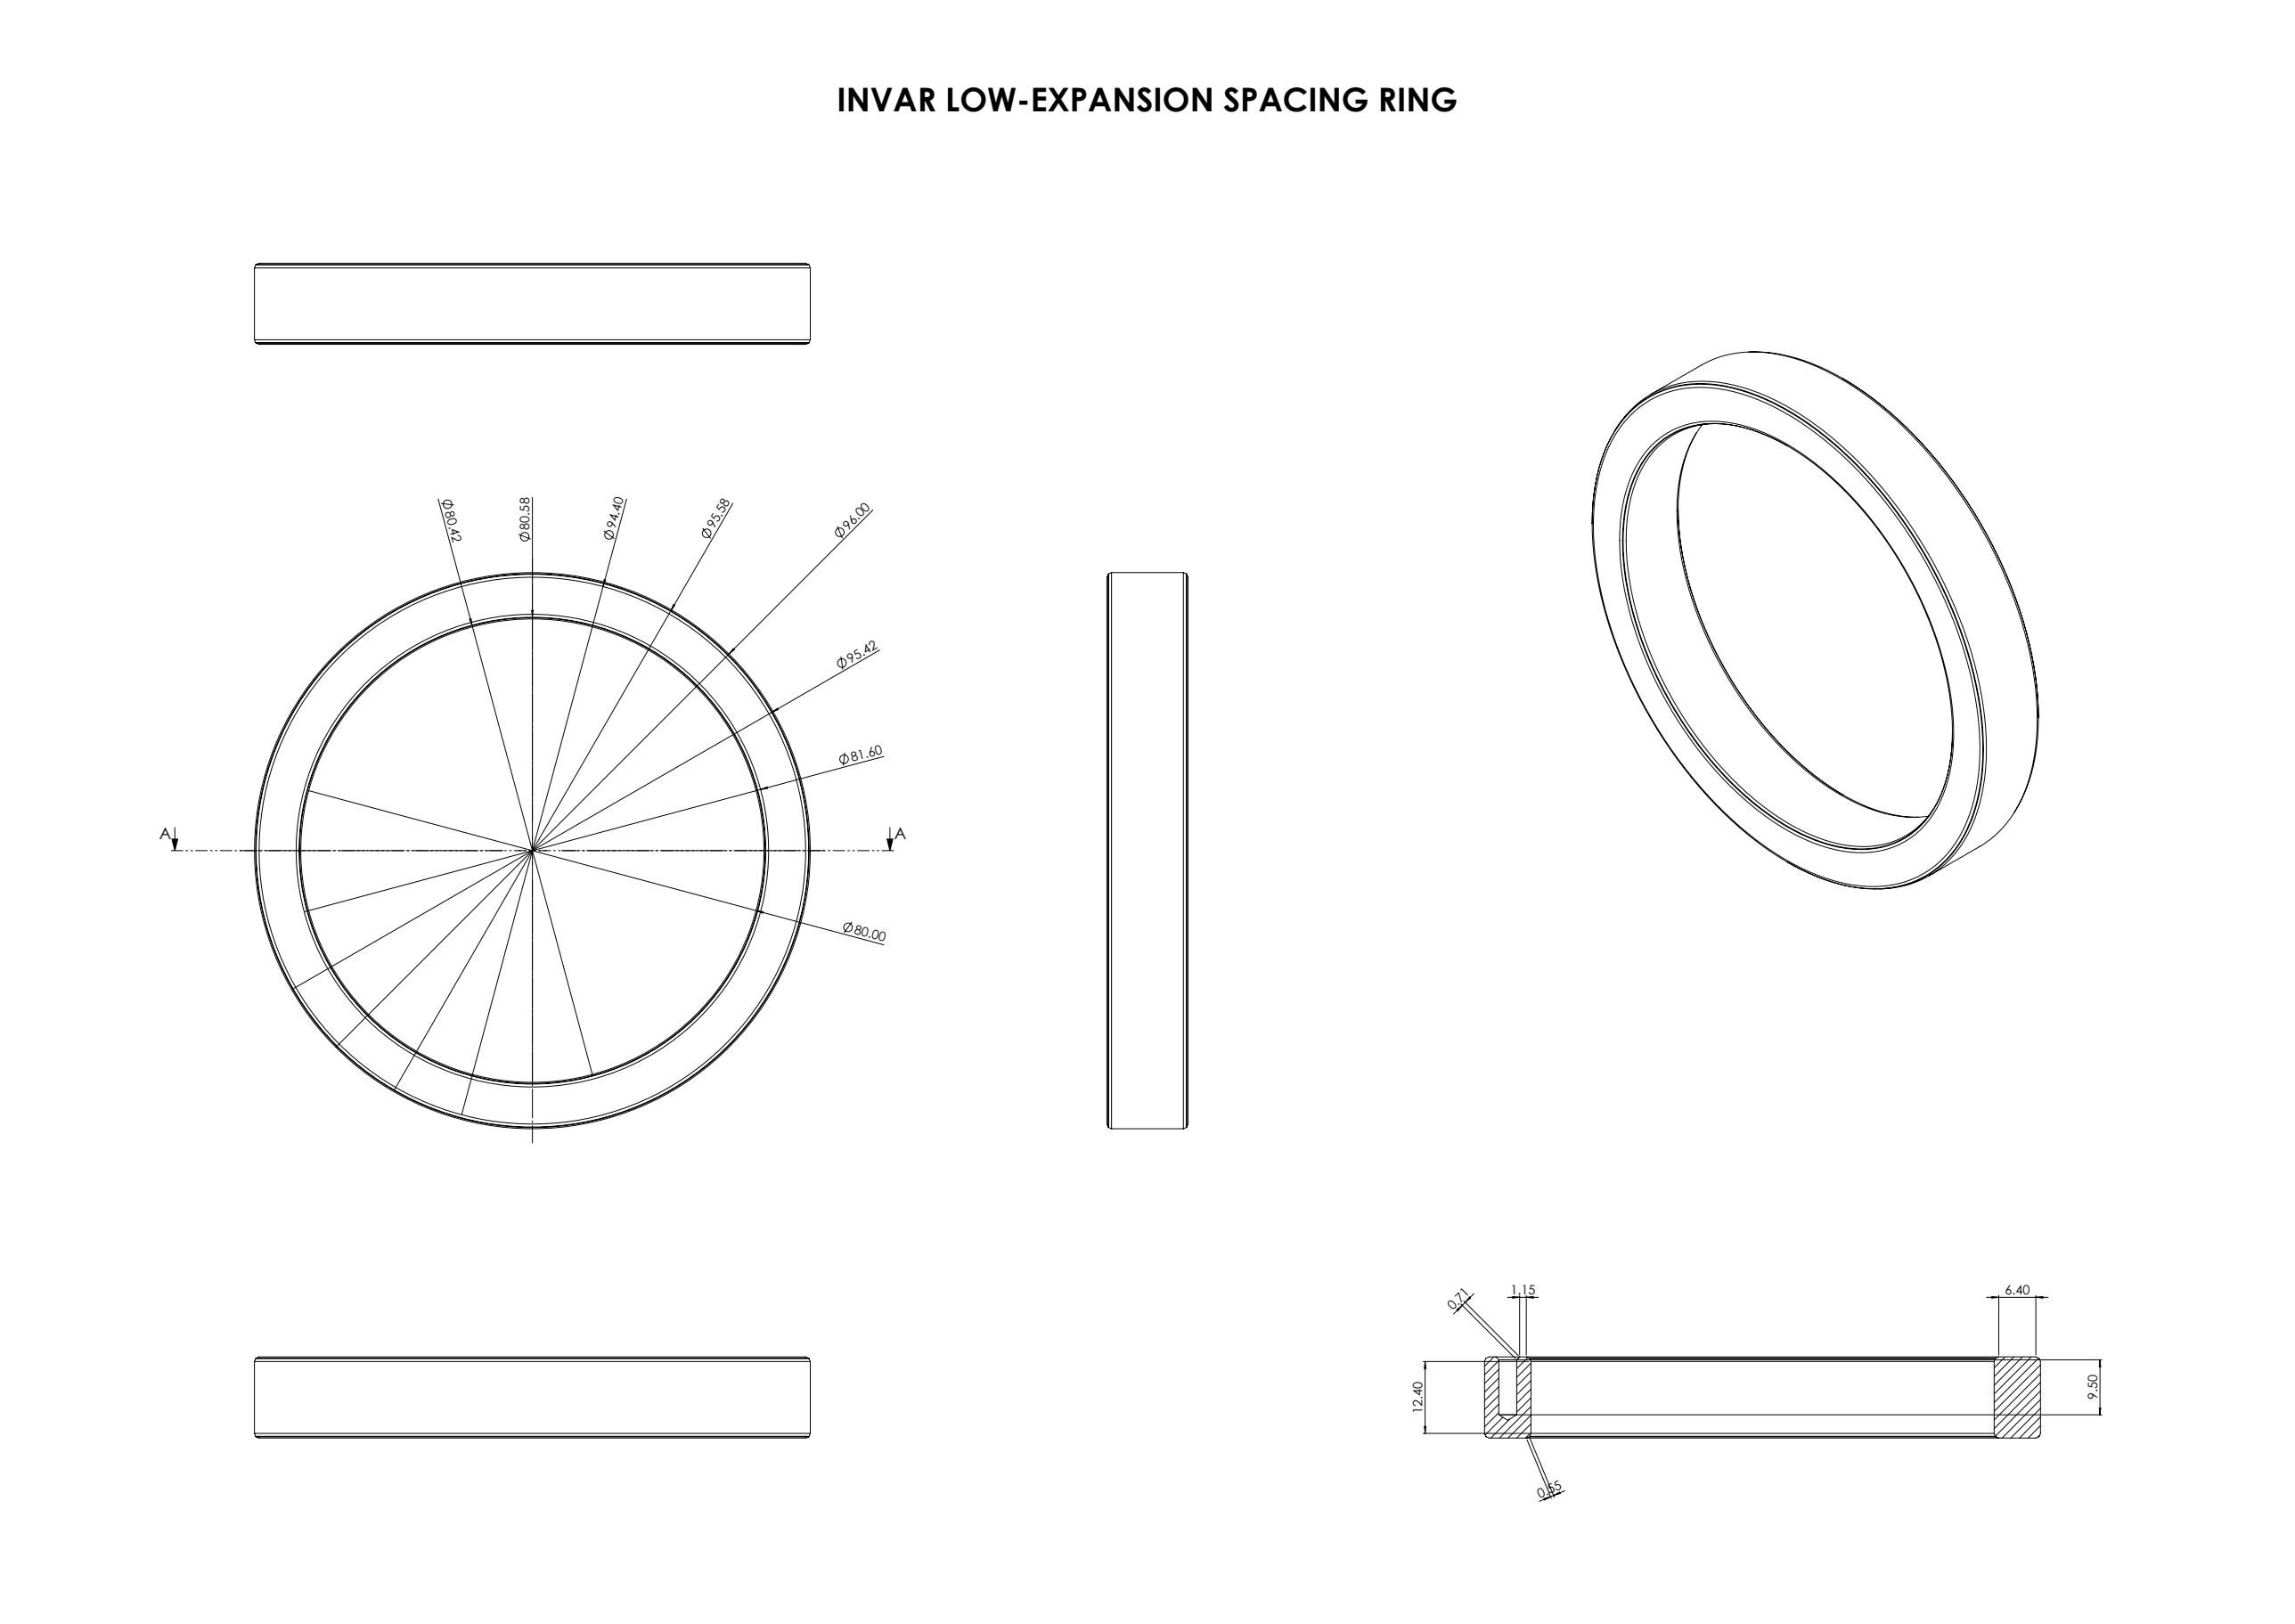
ISO-10303-21;
HEADER;
/* Generated by software containing ST-Developer
 * from STEP Tools, Inc. (www.steptools.com) 
 */

FILE_DESCRIPTION(
/* description */ (''),
/* implementation_level */ '2;1');

FILE_NAME(
/* name */ '04_Invar_Low-Expansion_Spacing_Ring.step',
/* time_stamp */ '2026-10-19T22:59:19-07:00',
/* author */ (''),
/* organization */ (''),
/* preprocessor_version */ 'ST-DEVELOPER v20.2',
/* originating_system */ 'Autodesk Translation Framework v15.15.0.0',
/* authorisation */ '');

FILE_SCHEMA (('AUTOMOTIVE_DESIGN { 1 0 10303 214 3 1 1 }'));
ENDSEC;

DATA;
#10=MECHANICAL_DESIGN_GEOMETRIC_PRESENTATION_REPRESENTATION('',(#914),#53650);
#882=SHAPE_REPRESENTATION_RELATIONSHIP('SRR','None',#53727,#898);
#898=ADVANCED_BREP_SHAPE_REPRESENTATION('',(#930),#53637);
#914=STYLED_ITEM('',(#53972),#930);
#930=MANIFOLD_SOLID_BREP('Invar Spacing Ring',#23306);
#987=CYLINDRICAL_SURFACE('',#23988,4.);
#988=CYLINDRICAL_SURFACE('',#24015,4.8);
#989=CYLINDRICAL_SURFACE('',#24025,0.155);
#990=CYLINDRICAL_SURFACE('',#24030,0.154999999999999);
#991=CYLINDRICAL_SURFACE('',#24035,0.155);
#1326=FACE_BOUND('',#3888,.T.);
#1327=FACE_BOUND('',#3889,.T.);
#1328=FACE_BOUND('',#3890,.T.);
#1329=FACE_BOUND('',#3891,.T.);
#1330=FACE_BOUND('',#3896,.T.);
#1549=PLANE('',#23999);
#1550=PLANE('',#24010);
#2504=FACE_OUTER_BOUND('',#3881,.T.);
#2505=FACE_OUTER_BOUND('',#3882,.T.);
#2506=FACE_OUTER_BOUND('',#3883,.T.);
#2507=FACE_OUTER_BOUND('',#3884,.T.);
#2508=FACE_OUTER_BOUND('',#3885,.T.);
#2509=FACE_OUTER_BOUND('',#3886,.T.);
#2510=FACE_OUTER_BOUND('',#3887,.T.);
#2511=FACE_OUTER_BOUND('',#3892,.T.);
#2512=FACE_OUTER_BOUND('',#3893,.T.);
#2513=FACE_OUTER_BOUND('',#3894,.T.);
#2514=FACE_OUTER_BOUND('',#3895,.T.);
#2515=FACE_OUTER_BOUND('',#3897,.T.);
#2516=FACE_OUTER_BOUND('',#3898,.T.);
#2517=FACE_OUTER_BOUND('',#3899,.T.);
#2518=FACE_OUTER_BOUND('',#3900,.T.);
#2519=FACE_OUTER_BOUND('',#3901,.T.);
#2520=FACE_OUTER_BOUND('',#3902,.T.);
#2521=FACE_OUTER_BOUND('',#3903,.T.);
#2522=FACE_OUTER_BOUND('',#3904,.T.);
#2523=FACE_OUTER_BOUND('',#3905,.T.);
#2524=FACE_OUTER_BOUND('',#3906,.T.);
#2525=FACE_OUTER_BOUND('',#3907,.T.);
#2526=FACE_OUTER_BOUND('',#3908,.T.);
#2527=FACE_OUTER_BOUND('',#3909,.T.);
#2528=FACE_OUTER_BOUND('',#3910,.T.);
#3881=EDGE_LOOP('',(#16211,#16212,#16213,#16214,#16215));
#3882=EDGE_LOOP('',(#16216,#16217,#16218,#16219,#16220,#16221));
#3883=EDGE_LOOP('',(#16222,#16223,#16224,#16225));
#3884=EDGE_LOOP('',(#16226,#16227,#16228,#16229,#16230));
#3885=EDGE_LOOP('',(#16231,#16232,#16233,#16234));
#3886=EDGE_LOOP('',(#16235,#16236,#16237,#16238));
#3887=EDGE_LOOP('',(#16239));
#3888=EDGE_LOOP('',(#16240));
#3889=EDGE_LOOP('',(#16241));
#3890=EDGE_LOOP('',(#16242));
#3891=EDGE_LOOP('',(#16243));
#3892=EDGE_LOOP('',(#16244,#16245,#16246,#16247));
#3893=EDGE_LOOP('',(#16248,#16249,#16250,#16251));
#3894=EDGE_LOOP('',(#16252,#16253,#16254,#16255));
#3895=EDGE_LOOP('',(#16256));
#3896=EDGE_LOOP('',(#16257));
#3897=EDGE_LOOP('',(#16258,#16259,#16260,#16261,#16262));
#3898=EDGE_LOOP('',(#16263,#16264,#16265,#16266,#16267,#16268));
#3899=EDGE_LOOP('',(#16269,#16270,#16271,#16272));
#3900=EDGE_LOOP('',(#16273,#16274,#16275,#16276));
#3901=EDGE_LOOP('',(#16277,#16278,#16279,#16280,#16281));
#3902=EDGE_LOOP('',(#16282,#16283,#16284));
#3903=EDGE_LOOP('',(#16285,#16286,#16287,#16288));
#3904=EDGE_LOOP('',(#16289,#16290,#16291,#16292));
#3905=EDGE_LOOP('',(#16293,#16294,#16295));
#3906=EDGE_LOOP('',(#16296,#16297,#16298,#16299));
#3907=EDGE_LOOP('',(#16300,#16301,#16302,#16303));
#3908=EDGE_LOOP('',(#16304,#16305,#16306));
#3909=EDGE_LOOP('',(#16307,#16308,#16309,#16310));
#3910=EDGE_LOOP('',(#16311,#16312,#16313,#16314));
#5278=CIRCLE('',#23985,4.0212132034356);
#5279=CIRCLE('',#23986,4.);
#5280=CIRCLE('',#23987,4.);
#5281=CIRCLE('',#23989,4.);
#5282=CIRCLE('',#23990,4.);
#5283=CIRCLE('',#23992,4.0287867965644);
#5284=CIRCLE('',#23994,4.0212132034356);
#5285=CIRCLE('',#23996,4.0287867965644);
#5286=CIRCLE('',#23998,4.08);
#5287=CIRCLE('',#24000,4.72);
#5288=CIRCLE('',#24001,0.205);
#5289=CIRCLE('',#24002,0.204999999999999);
#5290=CIRCLE('',#24003,0.205);
#5291=CIRCLE('',#24005,4.7712132034356);
#5292=CIRCLE('',#24007,4.7787867965644);
#5293=CIRCLE('',#24009,4.08);
#5294=CIRCLE('',#24011,4.72);
#5295=CIRCLE('',#24013,4.8);
#5296=CIRCLE('',#24014,4.8);
#5297=CIRCLE('',#24016,4.8);
#5298=CIRCLE('',#24017,4.8);
#5299=CIRCLE('',#24019,4.7712132034356);
#5300=CIRCLE('',#24021,4.7787867965644);
#5301=CIRCLE('',#24024,0.155);
#5302=CIRCLE('',#24026,0.155);
#5303=CIRCLE('',#24029,0.154999999999999);
#5304=CIRCLE('',#24031,0.154999999999999);
#5305=CIRCLE('',#24034,0.155);
#5306=CIRCLE('',#24036,0.155);
#6209=LINE('',#32993,#8054);
#6210=LINE('',#32999,#8055);
#6211=LINE('',#33005,#8056);
#6212=LINE('',#33010,#8057);
#6213=LINE('',#33014,#8058);
#6214=LINE('',#33017,#8059);
#6215=LINE('',#33031,#8060);
#6216=LINE('',#33035,#8061);
#6217=LINE('',#33038,#8062);
#6218=LINE('',#33045,#8063);
#6219=LINE('',#33054,#8064);
#6220=LINE('',#33058,#8065);
#6221=LINE('',#33061,#8066);
#6222=LINE('',#33064,#8067);
#6223=LINE('',#33068,#8068);
#6224=LINE('',#33072,#8069);
#6225=LINE('',#33075,#8070);
#6226=LINE('',#33079,#8071);
#6227=LINE('',#33083,#8072);
#6228=LINE('',#33086,#8073);
#6229=LINE('',#33090,#8074);
#6230=LINE('',#33094,#8075);
#6231=LINE('',#33097,#8076);
#8054=VECTOR('',#26991,4.0106066017178);
#8055=VECTOR('',#26998,4.);
#8056=VECTOR('',#27005,4.025);
#8057=VECTOR('',#27012,4.0106066017178);
#8058=VECTOR('',#27017,4.025);
#8059=VECTOR('',#27020,4.0543933982822);
#8060=VECTOR('',#27037,4.7456066017178);
#8061=VECTOR('',#27042,4.775);
#8062=VECTOR('',#27045,4.0543933982822);
#8063=VECTOR('',#27054,4.7893933982822);
#8064=VECTOR('',#27065,4.8);
#8065=VECTOR('',#27070,4.7456066017178);
#8066=VECTOR('',#27073,4.775);
#8067=VECTOR('',#27078,4.7893933982822);
#8068=VECTOR('',#27081,0.0774999999999997);
#8069=VECTOR('',#27086,0.155);
#8070=VECTOR('',#27091,0.205);
#8071=VECTOR('',#27094,0.0774999999999997);
#8072=VECTOR('',#27099,0.154999999999999);
#8073=VECTOR('',#27104,0.204999999999999);
#8074=VECTOR('',#27107,0.0774999999999997);
#8075=VECTOR('',#27112,0.155);
#8076=VECTOR('',#27117,0.205);
#9871=VERTEX_POINT('',#32990);
#9872=VERTEX_POINT('',#32992);
#9873=VERTEX_POINT('',#32994);
#9874=VERTEX_POINT('',#32998);
#9875=VERTEX_POINT('',#33000);
#9876=VERTEX_POINT('',#33004);
#9877=VERTEX_POINT('',#33008);
#9878=VERTEX_POINT('',#33012);
#9879=VERTEX_POINT('',#33016);
#9880=VERTEX_POINT('',#33020);
#9881=VERTEX_POINT('',#33022);
#9882=VERTEX_POINT('',#33024);
#9883=VERTEX_POINT('',#33026);
#9884=VERTEX_POINT('',#33029);
#9885=VERTEX_POINT('',#33033);
#9886=VERTEX_POINT('',#33037);
#9887=VERTEX_POINT('',#33041);
#9888=VERTEX_POINT('',#33044);
#9889=VERTEX_POINT('',#33046);
#9890=VERTEX_POINT('',#33050);
#9891=VERTEX_POINT('',#33051);
#9892=VERTEX_POINT('',#33056);
#9893=VERTEX_POINT('',#33060);
#9894=VERTEX_POINT('',#33066);
#9895=VERTEX_POINT('',#33067);
#9896=VERTEX_POINT('',#33071);
#9897=VERTEX_POINT('',#33077);
#9898=VERTEX_POINT('',#33078);
#9899=VERTEX_POINT('',#33082);
#9900=VERTEX_POINT('',#33088);
#9901=VERTEX_POINT('',#33089);
#9902=VERTEX_POINT('',#33093);
#12283=EDGE_CURVE('',#9871,#9871,#5278,.T.);
#12284=EDGE_CURVE('',#9871,#9872,#6209,.T.);
#12285=EDGE_CURVE('',#9872,#9873,#5279,.T.);
#12286=EDGE_CURVE('',#9873,#9872,#5280,.T.);
#12287=EDGE_CURVE('',#9873,#9874,#6210,.T.);
#12288=EDGE_CURVE('',#9875,#9874,#5281,.T.);
#12289=EDGE_CURVE('',#9874,#9875,#5282,.T.);
#12290=EDGE_CURVE('',#9871,#9876,#6211,.T.);
#12291=EDGE_CURVE('',#9876,#9876,#5283,.T.);
#12292=EDGE_CURVE('',#9877,#9877,#5284,.T.);
#12293=EDGE_CURVE('',#9877,#9875,#6212,.T.);
#12294=EDGE_CURVE('',#9878,#9878,#5285,.T.);
#12295=EDGE_CURVE('',#9878,#9877,#6213,.T.);
#12296=EDGE_CURVE('',#9878,#9879,#6214,.T.);
#12297=EDGE_CURVE('',#9879,#9879,#5286,.T.);
#12298=EDGE_CURVE('',#9880,#9880,#5287,.T.);
#12299=EDGE_CURVE('',#9881,#9881,#5288,.T.);
#12300=EDGE_CURVE('',#9882,#9882,#5289,.T.);
#12301=EDGE_CURVE('',#9883,#9883,#5290,.T.);
#12302=EDGE_CURVE('',#9884,#9884,#5291,.T.);
#12303=EDGE_CURVE('',#9884,#9880,#6215,.T.);
#12304=EDGE_CURVE('',#9885,#9885,#5292,.T.);
#12305=EDGE_CURVE('',#9885,#9884,#6216,.T.);
#12306=EDGE_CURVE('',#9876,#9886,#6217,.T.);
#12307=EDGE_CURVE('',#9886,#9886,#5293,.T.);
#12308=EDGE_CURVE('',#9887,#9887,#5294,.T.);
#12309=EDGE_CURVE('',#9885,#9888,#6218,.T.);
#12310=EDGE_CURVE('',#9888,#9889,#5295,.T.);
#12311=EDGE_CURVE('',#9889,#9888,#5296,.T.);
#12312=EDGE_CURVE('',#9890,#9891,#5297,.T.);
#12313=EDGE_CURVE('',#9891,#9890,#5298,.T.);
#12314=EDGE_CURVE('',#9891,#9889,#6219,.T.);
#12315=EDGE_CURVE('',#9892,#9892,#5299,.T.);
#12316=EDGE_CURVE('',#9892,#9887,#6220,.T.);
#12317=EDGE_CURVE('',#9892,#9893,#6221,.T.);
#12318=EDGE_CURVE('',#9893,#9893,#5300,.T.);
#12319=EDGE_CURVE('',#9893,#9890,#6222,.T.);
#12320=EDGE_CURVE('',#9894,#9895,#6223,.T.);
#12321=EDGE_CURVE('',#9895,#9895,#5301,.T.);
#12322=EDGE_CURVE('',#9895,#9896,#6224,.T.);
#12323=EDGE_CURVE('',#9896,#9896,#5302,.T.);
#12324=EDGE_CURVE('',#9896,#9881,#6225,.T.);
#12325=EDGE_CURVE('',#9897,#9898,#6226,.T.);
#12326=EDGE_CURVE('',#9898,#9898,#5303,.T.);
#12327=EDGE_CURVE('',#9898,#9899,#6227,.T.);
#12328=EDGE_CURVE('',#9899,#9899,#5304,.T.);
#12329=EDGE_CURVE('',#9899,#9882,#6228,.T.);
#12330=EDGE_CURVE('',#9900,#9901,#6229,.T.);
#12331=EDGE_CURVE('',#9901,#9901,#5305,.T.);
#12332=EDGE_CURVE('',#9901,#9902,#6230,.T.);
#12333=EDGE_CURVE('',#9902,#9902,#5306,.T.);
#12334=EDGE_CURVE('',#9902,#9883,#6231,.T.);
#16211=ORIENTED_EDGE('',*,*,#12283,.T.);
#16212=ORIENTED_EDGE('',*,*,#12284,.T.);
#16213=ORIENTED_EDGE('',*,*,#12285,.T.);
#16214=ORIENTED_EDGE('',*,*,#12286,.T.);
#16215=ORIENTED_EDGE('',*,*,#12284,.F.);
#16216=ORIENTED_EDGE('',*,*,#12285,.F.);
#16217=ORIENTED_EDGE('',*,*,#12286,.F.);
#16218=ORIENTED_EDGE('',*,*,#12287,.T.);
#16219=ORIENTED_EDGE('',*,*,#12288,.F.);
#16220=ORIENTED_EDGE('',*,*,#12289,.F.);
#16221=ORIENTED_EDGE('',*,*,#12287,.F.);
#16222=ORIENTED_EDGE('',*,*,#12283,.F.);
#16223=ORIENTED_EDGE('',*,*,#12290,.T.);
#16224=ORIENTED_EDGE('',*,*,#12291,.F.);
#16225=ORIENTED_EDGE('',*,*,#12290,.F.);
#16226=ORIENTED_EDGE('',*,*,#12292,.T.);
#16227=ORIENTED_EDGE('',*,*,#12293,.T.);
#16228=ORIENTED_EDGE('',*,*,#12288,.T.);
#16229=ORIENTED_EDGE('',*,*,#12289,.T.);
#16230=ORIENTED_EDGE('',*,*,#12293,.F.);
#16231=ORIENTED_EDGE('',*,*,#12294,.F.);
#16232=ORIENTED_EDGE('',*,*,#12295,.T.);
#16233=ORIENTED_EDGE('',*,*,#12292,.F.);
#16234=ORIENTED_EDGE('',*,*,#12295,.F.);
#16235=ORIENTED_EDGE('',*,*,#12294,.T.);
#16236=ORIENTED_EDGE('',*,*,#12296,.T.);
#16237=ORIENTED_EDGE('',*,*,#12297,.T.);
#16238=ORIENTED_EDGE('',*,*,#12296,.F.);
#16239=ORIENTED_EDGE('',*,*,#12298,.F.);
#16240=ORIENTED_EDGE('',*,*,#12299,.T.);
#16241=ORIENTED_EDGE('',*,*,#12300,.T.);
#16242=ORIENTED_EDGE('',*,*,#12301,.T.);
#16243=ORIENTED_EDGE('',*,*,#12297,.F.);
#16244=ORIENTED_EDGE('',*,*,#12302,.T.);
#16245=ORIENTED_EDGE('',*,*,#12303,.T.);
#16246=ORIENTED_EDGE('',*,*,#12298,.T.);
#16247=ORIENTED_EDGE('',*,*,#12303,.F.);
#16248=ORIENTED_EDGE('',*,*,#12304,.F.);
#16249=ORIENTED_EDGE('',*,*,#12305,.T.);
#16250=ORIENTED_EDGE('',*,*,#12302,.F.);
#16251=ORIENTED_EDGE('',*,*,#12305,.F.);
#16252=ORIENTED_EDGE('',*,*,#12291,.T.);
#16253=ORIENTED_EDGE('',*,*,#12306,.T.);
#16254=ORIENTED_EDGE('',*,*,#12307,.T.);
#16255=ORIENTED_EDGE('',*,*,#12306,.F.);
#16256=ORIENTED_EDGE('',*,*,#12308,.F.);
#16257=ORIENTED_EDGE('',*,*,#12307,.F.);
#16258=ORIENTED_EDGE('',*,*,#12304,.T.);
#16259=ORIENTED_EDGE('',*,*,#12309,.T.);
#16260=ORIENTED_EDGE('',*,*,#12310,.T.);
#16261=ORIENTED_EDGE('',*,*,#12311,.T.);
#16262=ORIENTED_EDGE('',*,*,#12309,.F.);
#16263=ORIENTED_EDGE('',*,*,#12312,.F.);
#16264=ORIENTED_EDGE('',*,*,#12313,.F.);
#16265=ORIENTED_EDGE('',*,*,#12314,.T.);
#16266=ORIENTED_EDGE('',*,*,#12310,.F.);
#16267=ORIENTED_EDGE('',*,*,#12311,.F.);
#16268=ORIENTED_EDGE('',*,*,#12314,.F.);
#16269=ORIENTED_EDGE('',*,*,#12315,.T.);
#16270=ORIENTED_EDGE('',*,*,#12316,.T.);
#16271=ORIENTED_EDGE('',*,*,#12308,.T.);
#16272=ORIENTED_EDGE('',*,*,#12316,.F.);
#16273=ORIENTED_EDGE('',*,*,#12315,.F.);
#16274=ORIENTED_EDGE('',*,*,#12317,.T.);
#16275=ORIENTED_EDGE('',*,*,#12318,.F.);
#16276=ORIENTED_EDGE('',*,*,#12317,.F.);
#16277=ORIENTED_EDGE('',*,*,#12318,.T.);
#16278=ORIENTED_EDGE('',*,*,#12319,.T.);
#16279=ORIENTED_EDGE('',*,*,#12312,.T.);
#16280=ORIENTED_EDGE('',*,*,#12313,.T.);
#16281=ORIENTED_EDGE('',*,*,#12319,.F.);
#16282=ORIENTED_EDGE('',*,*,#12320,.T.);
#16283=ORIENTED_EDGE('',*,*,#12321,.T.);
#16284=ORIENTED_EDGE('',*,*,#12320,.F.);
#16285=ORIENTED_EDGE('',*,*,#12321,.F.);
#16286=ORIENTED_EDGE('',*,*,#12322,.T.);
#16287=ORIENTED_EDGE('',*,*,#12323,.T.);
#16288=ORIENTED_EDGE('',*,*,#12322,.F.);
#16289=ORIENTED_EDGE('',*,*,#12323,.F.);
#16290=ORIENTED_EDGE('',*,*,#12324,.T.);
#16291=ORIENTED_EDGE('',*,*,#12299,.F.);
#16292=ORIENTED_EDGE('',*,*,#12324,.F.);
#16293=ORIENTED_EDGE('',*,*,#12325,.T.);
#16294=ORIENTED_EDGE('',*,*,#12326,.T.);
#16295=ORIENTED_EDGE('',*,*,#12325,.F.);
#16296=ORIENTED_EDGE('',*,*,#12326,.F.);
#16297=ORIENTED_EDGE('',*,*,#12327,.T.);
#16298=ORIENTED_EDGE('',*,*,#12328,.T.);
#16299=ORIENTED_EDGE('',*,*,#12327,.F.);
#16300=ORIENTED_EDGE('',*,*,#12328,.F.);
#16301=ORIENTED_EDGE('',*,*,#12329,.T.);
#16302=ORIENTED_EDGE('',*,*,#12300,.F.);
#16303=ORIENTED_EDGE('',*,*,#12329,.F.);
#16304=ORIENTED_EDGE('',*,*,#12330,.T.);
#16305=ORIENTED_EDGE('',*,*,#12331,.T.);
#16306=ORIENTED_EDGE('',*,*,#12330,.F.);
#16307=ORIENTED_EDGE('',*,*,#12331,.F.);
#16308=ORIENTED_EDGE('',*,*,#12332,.T.);
#16309=ORIENTED_EDGE('',*,*,#12333,.T.);
#16310=ORIENTED_EDGE('',*,*,#12332,.F.);
#16311=ORIENTED_EDGE('',*,*,#12333,.F.);
#16312=ORIENTED_EDGE('',*,*,#12334,.T.);
#16313=ORIENTED_EDGE('',*,*,#12301,.F.);
#16314=ORIENTED_EDGE('',*,*,#12334,.F.);
#21902=CONICAL_SURFACE('',#23984,4.0106066017178,0.392699081698746);
#21903=CONICAL_SURFACE('',#23991,4.025,0.785398163397446);
#21904=CONICAL_SURFACE('',#23993,4.0106066017178,0.392699081698729);
#21905=CONICAL_SURFACE('',#23995,4.025,0.785398163397446);
#21906=CONICAL_SURFACE('',#23997,4.0543933982822,1.17809724509616);
#21907=CONICAL_SURFACE('',#24004,4.7456066017178,1.17809724509618);
#21908=CONICAL_SURFACE('',#24006,4.775,0.785398163397446);
#21909=CONICAL_SURFACE('',#24008,4.0543933982822,1.17809724509617);
#21910=CONICAL_SURFACE('',#24012,4.7893933982822,0.392699081698714);
#21911=CONICAL_SURFACE('',#24018,4.7456066017178,1.17809724509618);
#21912=CONICAL_SURFACE('',#24020,4.775,0.785398163397446);
#21913=CONICAL_SURFACE('',#24022,4.7893933982822,0.392699081698714);
#21914=CONICAL_SURFACE('',#24023,0.0774999999999997,1.02974425867665);
#21915=CONICAL_SURFACE('',#24027,0.205,0.785398163397449);
#21916=CONICAL_SURFACE('',#24028,0.0774999999999997,1.02974425867665);
#21917=CONICAL_SURFACE('',#24032,0.204999999999999,0.785398163397447);
#21918=CONICAL_SURFACE('',#24033,0.0774999999999997,1.02974425867665);
#21919=CONICAL_SURFACE('',#24037,0.205,0.785398163397449);
#22243=ADVANCED_FACE('',(#2504),#21902,.F.);
#22244=ADVANCED_FACE('',(#2505),#987,.F.);
#22245=ADVANCED_FACE('',(#2506),#21903,.F.);
#22246=ADVANCED_FACE('',(#2507),#21904,.F.);
#22247=ADVANCED_FACE('',(#2508),#21905,.F.);
#22248=ADVANCED_FACE('',(#2509),#21906,.F.);
#22249=ADVANCED_FACE('',(#2510,#1326,#1327,#1328,#1329),#1549,.T.);
#22250=ADVANCED_FACE('',(#2511),#21907,.T.);
#22251=ADVANCED_FACE('',(#2512),#21908,.T.);
#22252=ADVANCED_FACE('',(#2513),#21909,.F.);
#22253=ADVANCED_FACE('',(#2514,#1330),#1550,.T.);
#22254=ADVANCED_FACE('',(#2515),#21910,.T.);
#22255=ADVANCED_FACE('',(#2516),#988,.T.);
#22256=ADVANCED_FACE('',(#2517),#21911,.T.);
#22257=ADVANCED_FACE('',(#2518),#21912,.T.);
#22258=ADVANCED_FACE('',(#2519),#21913,.T.);
#22259=ADVANCED_FACE('',(#2520),#21914,.F.);
#22260=ADVANCED_FACE('',(#2521),#989,.F.);
#22261=ADVANCED_FACE('',(#2522),#21915,.F.);
#22262=ADVANCED_FACE('',(#2523),#21916,.F.);
#22263=ADVANCED_FACE('',(#2524),#990,.F.);
#22264=ADVANCED_FACE('',(#2525),#21917,.F.);
#22265=ADVANCED_FACE('',(#2526),#21918,.F.);
#22266=ADVANCED_FACE('',(#2527),#991,.F.);
#22267=ADVANCED_FACE('',(#2528),#21919,.F.);
#23306=CLOSED_SHELL('',(#22243,#22244,#22245,#22246,#22247,#22248,#22249,
#22250,#22251,#22252,#22253,#22254,#22255,#22256,#22257,#22258,#22259,#22260,
#22261,#22262,#22263,#22264,#22265,#22266,#22267));
#23983=AXIS2_PLACEMENT_3D('',#32988,#26985,#26986);
#23984=AXIS2_PLACEMENT_3D('',#32989,#26987,#26988);
#23985=AXIS2_PLACEMENT_3D('',#32991,#26989,#26990);
#23986=AXIS2_PLACEMENT_3D('',#32995,#26992,#26993);
#23987=AXIS2_PLACEMENT_3D('',#32996,#26994,#26995);
#23988=AXIS2_PLACEMENT_3D('',#32997,#26996,#26997);
#23989=AXIS2_PLACEMENT_3D('',#33001,#26999,#27000);
#23990=AXIS2_PLACEMENT_3D('',#33002,#27001,#27002);
#23991=AXIS2_PLACEMENT_3D('',#33003,#27003,#27004);
#23992=AXIS2_PLACEMENT_3D('',#33006,#27006,#27007);
#23993=AXIS2_PLACEMENT_3D('',#33007,#27008,#27009);
#23994=AXIS2_PLACEMENT_3D('',#33009,#27010,#27011);
#23995=AXIS2_PLACEMENT_3D('',#33011,#27013,#27014);
#23996=AXIS2_PLACEMENT_3D('',#33013,#27015,#27016);
#23997=AXIS2_PLACEMENT_3D('',#33015,#27018,#27019);
#23998=AXIS2_PLACEMENT_3D('',#33018,#27021,#27022);
#23999=AXIS2_PLACEMENT_3D('',#33019,#27023,#27024);
#24000=AXIS2_PLACEMENT_3D('',#33021,#27025,#27026);
#24001=AXIS2_PLACEMENT_3D('',#33023,#27027,#27028);
#24002=AXIS2_PLACEMENT_3D('',#33025,#27029,#27030);
#24003=AXIS2_PLACEMENT_3D('',#33027,#27031,#27032);
#24004=AXIS2_PLACEMENT_3D('',#33028,#27033,#27034);
#24005=AXIS2_PLACEMENT_3D('',#33030,#27035,#27036);
#24006=AXIS2_PLACEMENT_3D('',#33032,#27038,#27039);
#24007=AXIS2_PLACEMENT_3D('',#33034,#27040,#27041);
#24008=AXIS2_PLACEMENT_3D('',#33036,#27043,#27044);
#24009=AXIS2_PLACEMENT_3D('',#33039,#27046,#27047);
#24010=AXIS2_PLACEMENT_3D('',#33040,#27048,#27049);
#24011=AXIS2_PLACEMENT_3D('',#33042,#27050,#27051);
#24012=AXIS2_PLACEMENT_3D('',#33043,#27052,#27053);
#24013=AXIS2_PLACEMENT_3D('',#33047,#27055,#27056);
#24014=AXIS2_PLACEMENT_3D('',#33048,#27057,#27058);
#24015=AXIS2_PLACEMENT_3D('',#33049,#27059,#27060);
#24016=AXIS2_PLACEMENT_3D('',#33052,#27061,#27062);
#24017=AXIS2_PLACEMENT_3D('',#33053,#27063,#27064);
#24018=AXIS2_PLACEMENT_3D('',#33055,#27066,#27067);
#24019=AXIS2_PLACEMENT_3D('',#33057,#27068,#27069);
#24020=AXIS2_PLACEMENT_3D('',#33059,#27071,#27072);
#24021=AXIS2_PLACEMENT_3D('',#33062,#27074,#27075);
#24022=AXIS2_PLACEMENT_3D('',#33063,#27076,#27077);
#24023=AXIS2_PLACEMENT_3D('',#33065,#27079,#27080);
#24024=AXIS2_PLACEMENT_3D('',#33069,#27082,#27083);
#24025=AXIS2_PLACEMENT_3D('',#33070,#27084,#27085);
#24026=AXIS2_PLACEMENT_3D('',#33073,#27087,#27088);
#24027=AXIS2_PLACEMENT_3D('',#33074,#27089,#27090);
#24028=AXIS2_PLACEMENT_3D('',#33076,#27092,#27093);
#24029=AXIS2_PLACEMENT_3D('',#33080,#27095,#27096);
#24030=AXIS2_PLACEMENT_3D('',#33081,#27097,#27098);
#24031=AXIS2_PLACEMENT_3D('',#33084,#27100,#27101);
#24032=AXIS2_PLACEMENT_3D('',#33085,#27102,#27103);
#24033=AXIS2_PLACEMENT_3D('',#33087,#27105,#27106);
#24034=AXIS2_PLACEMENT_3D('',#33091,#27108,#27109);
#24035=AXIS2_PLACEMENT_3D('',#33092,#27110,#27111);
#24036=AXIS2_PLACEMENT_3D('',#33095,#27113,#27114);
#24037=AXIS2_PLACEMENT_3D('',#33096,#27115,#27116);
#26985=DIRECTION('axis',(0.,0.,1.));
#26986=DIRECTION('refdir',(1.,0.,0.));
#26987=DIRECTION('center_axis',(0.,-4.80790650449101E-15,1.));
#26988=DIRECTION('ref_axis',(-1.,3.06971386583218E-17,0.));
#26989=DIRECTION('center_axis',(0.,0.,1.));
#26990=DIRECTION('ref_axis',(-1.,6.12323399573677E-17,0.));
#26991=DIRECTION('',(-0.38268343236511,4.40680849605938E-15,-0.923879532511278));
#26992=DIRECTION('center_axis',(0.,0.,-1.));
#26993=DIRECTION('ref_axis',(-1.,0.,0.));
#26994=DIRECTION('center_axis',(0.,0.,-1.));
#26995=DIRECTION('ref_axis',(-1.,0.,0.));
#26996=DIRECTION('center_axis',(0.,0.,1.));
#26997=DIRECTION('ref_axis',(1.,0.,0.));
#26998=DIRECTION('',(0.,0.,-1.));
#26999=DIRECTION('center_axis',(0.,0.,1.));
#27000=DIRECTION('ref_axis',(-1.,0.,0.));
#27001=DIRECTION('center_axis',(0.,0.,1.));
#27002=DIRECTION('ref_axis',(-1.,0.,0.));
#27003=DIRECTION('center_axis',(0.,0.,1.));
#27004=DIRECTION('ref_axis',(-1.,0.,0.));
#27005=DIRECTION('',(0.707106781186546,-8.65956056235492E-17,0.707106781186549));
#27006=DIRECTION('center_axis',(0.,0.,-1.));
#27007=DIRECTION('ref_axis',(-1.,6.12323399573677E-17,0.));
#27008=DIRECTION('center_axis',(0.,-4.80790650449097E-15,-1.));
#27009=DIRECTION('ref_axis',(-1.,3.06971386583218E-17,0.));
#27010=DIRECTION('center_axis',(0.,0.,-1.));
#27011=DIRECTION('ref_axis',(-1.,6.12323399573677E-17,0.));
#27012=DIRECTION('',(-0.382683432365094,4.5005389041659E-15,0.923879532511285));
#27013=DIRECTION('center_axis',(0.,0.,-1.));
#27014=DIRECTION('ref_axis',(-1.,0.,0.));
#27015=DIRECTION('center_axis',(0.,0.,1.));
#27016=DIRECTION('ref_axis',(-1.,6.12323399573677E-17,0.));
#27017=DIRECTION('',(-0.707106781186546,8.65956056235492E-17,0.707106781186549));
#27018=DIRECTION('center_axis',(0.,1.16291744192215E-14,-1.));
#27019=DIRECTION('ref_axis',(-1.,3.04228054001255E-17,0.));
#27020=DIRECTION('',(0.923879532511283,4.53532798631812E-15,-0.382683432365099));
#27021=DIRECTION('center_axis',(0.,0.,-1.));
#27022=DIRECTION('ref_axis',(-1.,0.,0.));
#27023=DIRECTION('center_axis',(0.,0.,-1.));
#27024=DIRECTION('ref_axis',(-1.,0.,0.));
#27025=DIRECTION('center_axis',(0.,0.,1.));
#27026=DIRECTION('ref_axis',(-1.,0.,0.));
#27027=DIRECTION('center_axis',(0.,0.,1.));
#27028=DIRECTION('ref_axis',(-1.,0.,0.));
#27029=DIRECTION('center_axis',(0.,0.,1.));
#27030=DIRECTION('ref_axis',(-1.,0.,0.));
#27031=DIRECTION('center_axis',(0.,0.,1.));
#27032=DIRECTION('ref_axis',(-1.,0.,0.));
#27033=DIRECTION('center_axis',(0.,1.37722032303527E-14,1.));
#27034=DIRECTION('ref_axis',(-1.,-3.078137037066E-17,0.));
#27035=DIRECTION('center_axis',(0.,0.,-1.));
#27036=DIRECTION('ref_axis',(-1.,-6.12323399573677E-17,0.));
#27037=DIRECTION('',(-0.923879532511289,-5.41197489271776E-15,-0.382683432365086));
#27038=DIRECTION('center_axis',(0.,0.,1.));
#27039=DIRECTION('ref_axis',(-1.,0.,0.));
#27040=DIRECTION('center_axis',(0.,0.,1.));
#27041=DIRECTION('ref_axis',(-1.,-6.12323399573676E-17,0.));
#27042=DIRECTION('',(-0.707106781186546,-8.65956056235491E-17,-0.707106781186549));
#27043=DIRECTION('center_axis',(0.,1.16291744192216E-14,1.));
#27044=DIRECTION('ref_axis',(-1.,3.04228054001255E-17,0.));
#27045=DIRECTION('',(0.923879532511284,4.30904276386059E-15,0.382683432365097));
#27046=DIRECTION('center_axis',(0.,0.,1.));
#27047=DIRECTION('ref_axis',(-1.,0.,0.));
#27048=DIRECTION('center_axis',(0.,0.,1.));
#27049=DIRECTION('ref_axis',(1.,0.,0.));
#27050=DIRECTION('center_axis',(0.,0.,-1.));
#27051=DIRECTION('ref_axis',(-1.,0.,0.));
#27052=DIRECTION('center_axis',(0.,-5.71368862092357E-15,1.));
#27053=DIRECTION('ref_axis',(-1.,-3.05483673377054E-17,0.));
#27054=DIRECTION('',(0.382683432365081,-5.31393482200127E-15,0.923879532511291));
#27055=DIRECTION('center_axis',(0.,0.,-1.));
#27056=DIRECTION('ref_axis',(-1.,0.,0.));
#27057=DIRECTION('center_axis',(0.,0.,-1.));
#27058=DIRECTION('ref_axis',(-1.,0.,0.));
#27059=DIRECTION('center_axis',(0.,0.,1.));
#27060=DIRECTION('ref_axis',(1.,0.,0.));
#27061=DIRECTION('center_axis',(0.,0.,1.));
#27062=DIRECTION('ref_axis',(-1.,0.,0.));
#27063=DIRECTION('center_axis',(0.,0.,1.));
#27064=DIRECTION('ref_axis',(-1.,0.,0.));
#27065=DIRECTION('',(0.,0.,-1.));
#27066=DIRECTION('center_axis',(0.,1.37722032303528E-14,-1.));
#27067=DIRECTION('ref_axis',(-1.,-3.078137037066E-17,0.));
#27068=DIRECTION('center_axis',(0.,0.,1.));
#27069=DIRECTION('ref_axis',(-1.,-6.12323399573677E-17,0.));
#27070=DIRECTION('',(-0.923879532511289,-5.18568967026023E-15,0.382683432365084));
#27071=DIRECTION('center_axis',(0.,0.,-1.));
#27072=DIRECTION('ref_axis',(-1.,0.,0.));
#27073=DIRECTION('',(0.707106781186546,8.65956056235491E-17,-0.707106781186549));
#27074=DIRECTION('center_axis',(0.,0.,-1.));
#27075=DIRECTION('ref_axis',(-1.,-6.12323399573677E-17,0.));
#27076=DIRECTION('center_axis',(0.,-5.71368862092356E-15,-1.));
#27077=DIRECTION('ref_axis',(-1.,-3.05483673377054E-17,0.));
#27078=DIRECTION('',(0.38268343236508,-5.22020441389474E-15,-0.923879532511291));
#27079=DIRECTION('center_axis',(0.,0.,-1.));
#27080=DIRECTION('ref_axis',(-1.,0.,0.));
#27081=DIRECTION('',(0.857167300702112,-1.04972719113862E-16,-0.515038074910055));
#27082=DIRECTION('center_axis',(0.,0.,-1.));
#27083=DIRECTION('ref_axis',(1.,0.,0.));
#27084=DIRECTION('center_axis',(0.,0.,-1.));
#27085=DIRECTION('ref_axis',(-1.,0.,0.));
#27086=DIRECTION('',(0.,0.,-1.));
#27087=DIRECTION('center_axis',(0.,0.,-1.));
#27088=DIRECTION('ref_axis',(1.,0.,0.));
#27089=DIRECTION('center_axis',(0.,0.,-1.));
#27090=DIRECTION('ref_axis',(-1.,0.,0.));
#27091=DIRECTION('',(0.707106781186548,-8.65956056235494E-17,-0.707106781186547));
#27092=DIRECTION('center_axis',(0.,0.,-1.));
#27093=DIRECTION('ref_axis',(-1.,0.,0.));
#27094=DIRECTION('',(0.857167300702111,-1.04972719113862E-16,-0.515038074910056));
#27095=DIRECTION('center_axis',(0.,0.,-1.));
#27096=DIRECTION('ref_axis',(1.,0.,0.));
#27097=DIRECTION('center_axis',(0.,0.,-1.));
#27098=DIRECTION('ref_axis',(-1.,0.,0.));
#27099=DIRECTION('',(0.,0.,-1.));
#27100=DIRECTION('center_axis',(0.,0.,-1.));
#27101=DIRECTION('ref_axis',(1.,0.,0.));
#27102=DIRECTION('center_axis',(0.,0.,-1.));
#27103=DIRECTION('ref_axis',(-1.,0.,0.));
#27104=DIRECTION('',(0.707106781186546,-8.65956056235492E-17,-0.707106781186549));
#27105=DIRECTION('center_axis',(0.,0.,-1.));
#27106=DIRECTION('ref_axis',(-1.,0.,0.));
#27107=DIRECTION('',(0.857167300702112,-1.04972719113862E-16,-0.515038074910055));
#27108=DIRECTION('center_axis',(0.,0.,-1.));
#27109=DIRECTION('ref_axis',(1.,0.,0.));
#27110=DIRECTION('center_axis',(0.,0.,-1.));
#27111=DIRECTION('ref_axis',(-1.,0.,0.));
#27112=DIRECTION('',(0.,0.,-1.));
#27113=DIRECTION('center_axis',(0.,0.,-1.));
#27114=DIRECTION('ref_axis',(1.,0.,0.));
#27115=DIRECTION('center_axis',(0.,0.,-1.));
#27116=DIRECTION('ref_axis',(-1.,0.,0.));
#27117=DIRECTION('',(0.707106781186548,-8.65956056235494E-17,-0.707106781186547));
#32988=CARTESIAN_POINT('',(0.,0.,0.));
#32989=CARTESIAN_POINT('Origin',(0.,-1.23114146956912E-16,1.3456066017178));
#32990=CARTESIAN_POINT('',(4.0212132034356,0.,1.3712132034356));
#32991=CARTESIAN_POINT('Origin',(0.,-2.46228293913824E-16,1.3712132034356));
#32992=CARTESIAN_POINT('',(4.,-4.89858719658941E-16,1.32));
#32993=CARTESIAN_POINT('',(4.0106066017178,2.44929359829471E-16,1.3456066017178));
#32994=CARTESIAN_POINT('',(-4.,-4.89858719658941E-16,1.32));
#32995=CARTESIAN_POINT('Origin',(0.,0.,1.32));
#32996=CARTESIAN_POINT('Origin',(0.,0.,1.32));
#32997=CARTESIAN_POINT('Origin',(0.,0.,0.7));
#32998=CARTESIAN_POINT('',(-4.,-4.89858719658941E-16,0.08));
#32999=CARTESIAN_POINT('',(-4.,-4.89858719658941E-16,0.7));
#33000=CARTESIAN_POINT('',(4.,4.89858719658941E-16,0.08));
#33001=CARTESIAN_POINT('Origin',(0.,0.,0.08));
#33002=CARTESIAN_POINT('Origin',(0.,0.,0.08));
#33003=CARTESIAN_POINT('Origin',(0.,0.,1.375));
#33004=CARTESIAN_POINT('',(4.0287867965644,-9.86768170971943E-16,1.3787867965644));
#33005=CARTESIAN_POINT('',(4.025,-4.9292033665681E-16,1.375));
#33006=CARTESIAN_POINT('Origin',(0.,-2.46692042742986E-16,1.3787867965644));
#33007=CARTESIAN_POINT('Origin',(0.,-1.23114146956912E-16,0.0543933982822017));
#33008=CARTESIAN_POINT('',(4.0212132034356,-9.84913175655296E-16,0.0287867965644034));
#33009=CARTESIAN_POINT('Origin',(0.,-2.46228293913824E-16,0.0287867965644034));
#33010=CARTESIAN_POINT('',(4.0106066017178,-7.37385947657118E-16,0.0543933982822017));
#33011=CARTESIAN_POINT('Origin',(0.,0.,0.025));
#33012=CARTESIAN_POINT('',(4.0287867965644,0.,0.0212132034355969));
#33013=CARTESIAN_POINT('Origin',(0.,-2.46692042742986E-16,0.0212132034355969));
#33014=CARTESIAN_POINT('',(4.025,-4.9292033665681E-16,0.025));
#33015=CARTESIAN_POINT('Origin',(0.,-1.23346021371493E-16,0.0106066017177984));
#33016=CARTESIAN_POINT('',(4.08,-4.9965589405212E-16,0.));
#33017=CARTESIAN_POINT('',(4.0543933982822,2.4982794702606E-16,0.0106066017177984));
#33018=CARTESIAN_POINT('Origin',(0.,0.,0.));
#33019=CARTESIAN_POINT('Origin',(4.8,0.,0.));
#33020=CARTESIAN_POINT('',(4.72,5.78033289197551E-16,0.));
#33021=CARTESIAN_POINT('Origin',(0.,0.,0.));
#33022=CARTESIAN_POINT('',(2.405,-3.81051177665153,0.));
#33023=CARTESIAN_POINT('Origin',(2.2,-3.81051177665153,0.));
#33024=CARTESIAN_POINT('',(-4.195,5.63949851007356E-16,0.));
#33025=CARTESIAN_POINT('Origin',(-4.4,5.38844591624835E-16,0.));
#33026=CARTESIAN_POINT('',(2.405,3.81051177665153,0.));
#33027=CARTESIAN_POINT('Origin',(2.2,3.81051177665153,0.));
#33028=CARTESIAN_POINT('Origin',(0.,1.46076274440925E-16,0.0106066017177982));
#33029=CARTESIAN_POINT('',(4.7712132034356,0.,0.0212132034355964));
#33030=CARTESIAN_POINT('Origin',(0.,2.9215254888185E-16,0.0212132034355964));
#33031=CARTESIAN_POINT('',(4.7456066017178,8.73321742362474E-16,0.0106066017177982));
#33032=CARTESIAN_POINT('Origin',(0.,0.,0.025));
#33033=CARTESIAN_POINT('',(4.7787867965644,1.17046519084405E-15,0.0287867965644034));
#33034=CARTESIAN_POINT('Origin',(0.,2.92616297711012E-16,0.0287867965644034));
#33035=CARTESIAN_POINT('',(4.775,5.84768846592861E-16,0.025));
#33036=CARTESIAN_POINT('Origin',(0.,-1.23346021371493E-16,1.3893933982822));
#33037=CARTESIAN_POINT('',(4.08,4.9965589405212E-16,1.4));
#33038=CARTESIAN_POINT('',(4.0543933982822,-7.43212032512032E-16,1.3893933982822));
#33039=CARTESIAN_POINT('Origin',(0.,0.,1.4));
#33040=CARTESIAN_POINT('Origin',(4.,0.,1.4));
#33041=CARTESIAN_POINT('',(4.72,-5.78033289197551E-16,1.4));
#33042=CARTESIAN_POINT('Origin',(0.,0.,1.4));
#33043=CARTESIAN_POINT('Origin',(0.,1.46308148855506E-16,0.0543933982822016));
#33044=CARTESIAN_POINT('',(4.8,-5.8783046359073E-16,0.0799999999999998));
#33045=CARTESIAN_POINT('',(4.7893933982822,-2.93915231795365E-16,0.0543933982822016));
#33046=CARTESIAN_POINT('',(-4.8,-5.8783046359073E-16,0.0799999999999997));
#33047=CARTESIAN_POINT('Origin',(0.,0.,0.0799999999999998));
#33048=CARTESIAN_POINT('Origin',(0.,0.,0.0799999999999998));
#33049=CARTESIAN_POINT('Origin',(0.,0.,0.7));
#33050=CARTESIAN_POINT('',(4.8,5.8783046359073E-16,1.32));
#33051=CARTESIAN_POINT('',(-4.8,-5.8783046359073E-16,1.32));
#33052=CARTESIAN_POINT('Origin',(0.,0.,1.32));
#33053=CARTESIAN_POINT('Origin',(0.,0.,1.32));
#33054=CARTESIAN_POINT('',(-4.8,-5.8783046359073E-16,0.7));
#33055=CARTESIAN_POINT('Origin',(0.,1.46076274440925E-16,1.3893933982822));
#33056=CARTESIAN_POINT('',(4.7712132034356,1.1686101955274E-15,1.3787867965644));
#33057=CARTESIAN_POINT('Origin',(0.,2.9215254888185E-16,1.3787867965644));
#33058=CARTESIAN_POINT('',(4.7456066017178,-2.89016644598775E-16,1.3893933982822));
#33059=CARTESIAN_POINT('Origin',(0.,0.,1.375));
#33060=CARTESIAN_POINT('',(4.7787867965644,0.,1.3712132034356));
#33061=CARTESIAN_POINT('',(4.775,5.84768846592861E-16,1.375));
#33062=CARTESIAN_POINT('Origin',(0.,2.92616297711012E-16,1.3712132034356));
#33063=CARTESIAN_POINT('Origin',(0.,1.46308148855506E-16,1.3456066017178));
#33064=CARTESIAN_POINT('',(4.7893933982822,8.79147827217388E-16,1.3456066017178));
#33065=CARTESIAN_POINT('Origin',(2.2,-3.81051177665153,1.04656669797464));
#33066=CARTESIAN_POINT('',(2.2,-3.81051177665153,1.09313339594927));
#33067=CARTESIAN_POINT('',(2.355,-3.81051177665153,1.));
#33068=CARTESIAN_POINT('',(2.2775,-3.81051177665153,1.04656669797464));
#33069=CARTESIAN_POINT('Origin',(2.2,-3.81051177665153,1.));
#33070=CARTESIAN_POINT('Origin',(2.2,-3.81051177665153,0.525));
#33071=CARTESIAN_POINT('',(2.355,-3.81051177665153,0.05));
#33072=CARTESIAN_POINT('',(2.355,-3.81051177665153,0.525));
#33073=CARTESIAN_POINT('Origin',(2.2,-3.81051177665153,0.05));
#33074=CARTESIAN_POINT('Origin',(2.2,-3.81051177665153,-6.93889390390723E-18));
#33075=CARTESIAN_POINT('',(2.405,-3.81051177665153,-6.93889390390723E-18));
#33076=CARTESIAN_POINT('Origin',(-4.4,5.38844591624835E-16,1.04656669797464));
#33077=CARTESIAN_POINT('',(-4.4,5.38844591624835E-16,1.09313339594927));
#33078=CARTESIAN_POINT('',(-4.245,5.19862566238052E-16,1.));
#33079=CARTESIAN_POINT('',(-4.3225,5.29353578931443E-16,1.04656669797464));
#33080=CARTESIAN_POINT('Origin',(-4.4,5.38844591624835E-16,1.));
#33081=CARTESIAN_POINT('Origin',(-4.4,5.38844591624835E-16,0.525));
#33082=CARTESIAN_POINT('',(-4.245,5.19862566238051E-16,0.05));
#33083=CARTESIAN_POINT('',(-4.245,5.19862566238051E-16,0.525));
#33084=CARTESIAN_POINT('Origin',(-4.4,5.38844591624835E-16,0.05));
#33085=CARTESIAN_POINT('Origin',(-4.4,5.38844591624835E-16,0.));
#33086=CARTESIAN_POINT('',(-4.195,5.13739332242315E-16,0.));
#33087=CARTESIAN_POINT('Origin',(2.2,3.81051177665153,1.04656669797464));
#33088=CARTESIAN_POINT('',(2.2,3.81051177665153,1.09313339594927));
#33089=CARTESIAN_POINT('',(2.355,3.81051177665153,1.));
#33090=CARTESIAN_POINT('',(2.2775,3.81051177665153,1.04656669797464));
#33091=CARTESIAN_POINT('Origin',(2.2,3.81051177665153,1.));
#33092=CARTESIAN_POINT('Origin',(2.2,3.81051177665153,0.525));
#33093=CARTESIAN_POINT('',(2.355,3.81051177665153,0.05));
#33094=CARTESIAN_POINT('',(2.355,3.81051177665153,0.525));
#33095=CARTESIAN_POINT('Origin',(2.2,3.81051177665153,0.05));
#33096=CARTESIAN_POINT('Origin',(2.2,3.81051177665153,-6.93889390390723E-18));
#33097=CARTESIAN_POINT('',(2.405,3.81051177665153,-6.93889390390723E-18));
#53619=UNCERTAINTY_MEASURE_WITH_UNIT(LENGTH_MEASURE(0.001),#53651,
'DISTANCE_ACCURACY_VALUE',
'Maximum model space distance between geometric entities at asserted c
onnectivities');
#53632=UNCERTAINTY_MEASURE_WITH_UNIT(LENGTH_MEASURE(0.001),#53651,
'DISTANCE_ACCURACY_VALUE',
'Maximum model space distance between geometric entities at asserted c
onnectivities');
#53637=(
GEOMETRIC_REPRESENTATION_CONTEXT(3)
GLOBAL_UNCERTAINTY_ASSIGNED_CONTEXT((#53619))
GLOBAL_UNIT_ASSIGNED_CONTEXT((#53651,#53653,#53654))
REPRESENTATION_CONTEXT('','3D')
);
#53650=(
GEOMETRIC_REPRESENTATION_CONTEXT(3)
GLOBAL_UNCERTAINTY_ASSIGNED_CONTEXT((#53632))
GLOBAL_UNIT_ASSIGNED_CONTEXT((#53651,#53653,#53654))
REPRESENTATION_CONTEXT('','3D')
);
#53651=(
LENGTH_UNIT()
NAMED_UNIT(*)
SI_UNIT(.CENTI.,.METRE.)
);
#53653=(
NAMED_UNIT(*)
PLANE_ANGLE_UNIT()
SI_UNIT($,.RADIAN.)
);
#53654=(
NAMED_UNIT(*)
SI_UNIT($,.STERADIAN.)
SOLID_ANGLE_UNIT()
);
#53659=SHAPE_DEFINITION_REPRESENTATION(#53676,#53727);
#53676=PRODUCT_DEFINITION_SHAPE('',$,#53745);
#53727=SHAPE_REPRESENTATION('',(#23983),#53637);
#53740=PRODUCT_DEFINITION_CONTEXT('part definition',#53793,'design');
#53745=PRODUCT_DEFINITION('2026-10-18-22-44-37-726',
'04_Invar_Low-Expansion_Spacing_Ring',#53762,#53740);
#53762=PRODUCT_DEFINITION_FORMATION('',$,#53799);
#53793=APPLICATION_CONTEXT(
'Core Data for Automotive Mechanical Design Process');
#53794=PRODUCT_CONTEXT('part definition',#53793,'mechanical');
#53799=PRODUCT('2026-10-18-22-44-37-726',
'04_Invar_Low-Expansion_Spacing_Ring',$,(#53794));
#53966=COLOUR_RGB('Off White',0.89,0.88,0.83);
#53967=FILL_AREA_STYLE_COLOUR('',#53966);
#53968=FILL_AREA_STYLE('',(#53967));
#53969=SURFACE_STYLE_FILL_AREA(#53968);
#53970=SURFACE_SIDE_STYLE('',(#53969));
#53971=SURFACE_STYLE_USAGE(.BOTH.,#53970);
#53972=PRESENTATION_STYLE_ASSIGNMENT((#53971));
ENDSEC;
END-ISO-10303-21;
